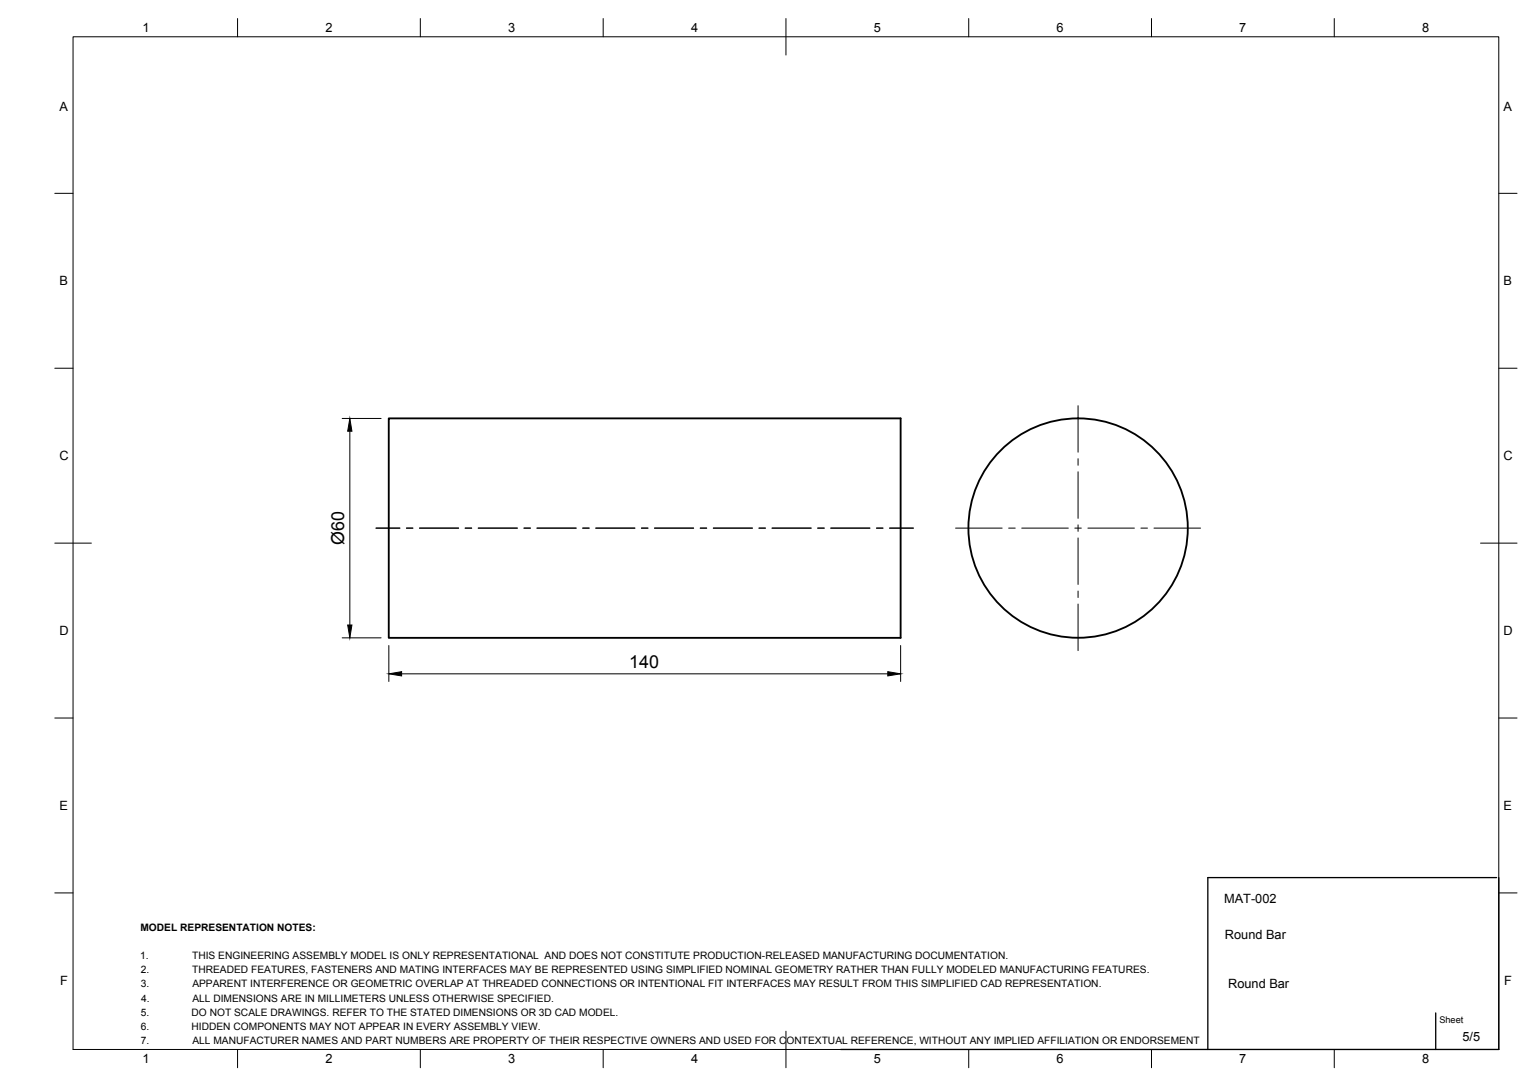
ISO-10303-21;
HEADER;
/* Generated by software containing ST-Developer
 * from STEP Tools, Inc. (www.steptools.com) 
 */

FILE_DESCRIPTION(
/* description */ ('STEP AP214'),
/* implementation_level */ '2;1');

FILE_NAME(
/* name */ 'Round Bar.step',
/* time_stamp */ '2026-11-14T04:35:10-08:00',
/* author */ (''),
/* organization */ (''),
/* preprocessor_version */ 'ST-DEVELOPER v20.2',
/* originating_system */ 'Autodesk Translation Framework v15.17.0.0',
/* authorisation */ '');

FILE_SCHEMA (('AUTOMOTIVE_DESIGN { 1 0 10303 214 3 1 1 }'));
ENDSEC;

DATA;
#10=MECHANICAL_DESIGN_GEOMETRIC_PRESENTATION_REPRESENTATION('',(#109),#2477);
#65=CIRCLE('',#1547,30.);
#66=CIRCLE('',#1548,30.);
#96=CYLINDRICAL_SURFACE('',#1546,30.);
#101=SHAPE_REPRESENTATION_RELATIONSHIP('SRR','None',#2499,#105);
#105=ADVANCED_BREP_SHAPE_REPRESENTATION('',(#113),#2475);
#109=STYLED_ITEM('',(#2528),#113);
#113=MANIFOLD_SOLID_BREP('Body1',#1429);
#166=FACE_OUTER_BOUND('',#247,.T.);
#167=FACE_OUTER_BOUND('',#248,.T.);
#168=FACE_OUTER_BOUND('',#249,.T.);
#247=EDGE_LOOP('',(#1178,#1179,#1180,#1181));
#248=EDGE_LOOP('',(#1182));
#249=EDGE_LOOP('',(#1183));
#401=LINE('',#2326,#548);
#548=VECTOR('',#1869,30.);
#665=VERTEX_POINT('',#2323);
#666=VERTEX_POINT('',#2325);
#839=EDGE_CURVE('',#665,#665,#65,.T.);
#840=EDGE_CURVE('',#665,#666,#401,.T.);
#841=EDGE_CURVE('',#666,#666,#66,.T.);
#1178=ORIENTED_EDGE('',*,*,#839,.F.);
#1179=ORIENTED_EDGE('',*,*,#840,.T.);
#1180=ORIENTED_EDGE('',*,*,#841,.T.);
#1181=ORIENTED_EDGE('',*,*,#840,.F.);
#1182=ORIENTED_EDGE('',*,*,#841,.F.);
#1183=ORIENTED_EDGE('',*,*,#839,.T.);
#1331=PLANE('',#1549);
#1332=PLANE('',#1550);
#1399=ADVANCED_FACE('',(#166),#96,.T.);
#1400=ADVANCED_FACE('',(#167),#1331,.F.);
#1401=ADVANCED_FACE('',(#168),#1332,.T.);
#1429=CLOSED_SHELL('',(#1399,#1400,#1401));
#1545=AXIS2_PLACEMENT_3D('',#2321,#1863,#1864);
#1546=AXIS2_PLACEMENT_3D('',#2322,#1865,#1866);
#1547=AXIS2_PLACEMENT_3D('',#2324,#1867,#1868);
#1548=AXIS2_PLACEMENT_3D('',#2327,#1870,#1871);
#1549=AXIS2_PLACEMENT_3D('',#2328,#1872,#1873);
#1550=AXIS2_PLACEMENT_3D('',#2329,#1874,#1875);
#1863=DIRECTION('axis',(0.,0.,1.));
#1864=DIRECTION('refdir',(1.,0.,0.));
#1865=DIRECTION('center_axis',(0.,0.,1.));
#1866=DIRECTION('ref_axis',(1.,0.,0.));
#1867=DIRECTION('center_axis',(0.,0.,1.));
#1868=DIRECTION('ref_axis',(1.,0.,0.));
#1869=DIRECTION('',(0.,0.,-1.));
#1870=DIRECTION('center_axis',(0.,0.,1.));
#1871=DIRECTION('ref_axis',(1.,0.,0.));
#1872=DIRECTION('center_axis',(0.,0.,1.));
#1873=DIRECTION('ref_axis',(1.,0.,0.));
#1874=DIRECTION('center_axis',(0.,0.,1.));
#1875=DIRECTION('ref_axis',(1.,0.,0.));
#2321=CARTESIAN_POINT('',(0.,0.,0.));
#2322=CARTESIAN_POINT('Origin',(-3.0679035930424E-16,0.,-105.));
#2323=CARTESIAN_POINT('',(-30.,-3.67394039744206E-15,35.));
#2324=CARTESIAN_POINT('Origin',(-3.0679035930424E-16,0.,35.));
#2325=CARTESIAN_POINT('',(-30.,-3.67394039744206E-15,-105.));
#2326=CARTESIAN_POINT('',(-30.,-3.67394039744206E-15,-105.));
#2327=CARTESIAN_POINT('Origin',(-3.0679035930424E-16,0.,-105.));
#2328=CARTESIAN_POINT('Origin',(-3.0679035930424E-16,0.,-105.));
#2329=CARTESIAN_POINT('Origin',(-3.0679035930424E-16,0.,35.));
#2469=UNCERTAINTY_MEASURE_WITH_UNIT(LENGTH_MEASURE(0.01),#2478,
'DISTANCE_ACCURACY_VALUE',
'Maximum model space distance between geometric entities at asserted c
onnectivities');
#2471=UNCERTAINTY_MEASURE_WITH_UNIT(LENGTH_MEASURE(0.01),#2478,
'DISTANCE_ACCURACY_VALUE',
'Maximum model space distance between geometric entities at asserted c
onnectivities');
#2475=(
GEOMETRIC_REPRESENTATION_CONTEXT(3)
GLOBAL_UNCERTAINTY_ASSIGNED_CONTEXT((#2469))
GLOBAL_UNIT_ASSIGNED_CONTEXT((#2478,#2480,#2481))
REPRESENTATION_CONTEXT('','3D')
);
#2477=(
GEOMETRIC_REPRESENTATION_CONTEXT(3)
GLOBAL_UNCERTAINTY_ASSIGNED_CONTEXT((#2471))
GLOBAL_UNIT_ASSIGNED_CONTEXT((#2478,#2480,#2481))
REPRESENTATION_CONTEXT('','3D')
);
#2478=(
LENGTH_UNIT()
NAMED_UNIT(*)
SI_UNIT(.MILLI.,.METRE.)
);
#2480=(
NAMED_UNIT(*)
PLANE_ANGLE_UNIT()
SI_UNIT($,.RADIAN.)
);
#2481=(
NAMED_UNIT(*)
SI_UNIT($,.STERADIAN.)
SOLID_ANGLE_UNIT()
);
#2485=SHAPE_DEFINITION_REPRESENTATION(#2490,#2499);
#2490=PRODUCT_DEFINITION_SHAPE('',$,#2505);
#2499=SHAPE_REPRESENTATION('',(#1545),#2475);
#2501=PRODUCT_DEFINITION_CONTEXT('part definition',#2518,'design');
#2505=PRODUCT_DEFINITION('Round Bar','Round Bar',#2510,#2501);
#2510=PRODUCT_DEFINITION_FORMATION('',$,#2523);
#2518=APPLICATION_CONTEXT(
'Core Data for Automotive Mechanical Design Process');
#2519=PRODUCT_CONTEXT('part definition',#2518,'mechanical');
#2523=PRODUCT('Round Bar','Round Bar',$,(#2519));
#2528=PRESENTATION_STYLE_ASSIGNMENT((#2533));
#2533=SURFACE_STYLE_USAGE(.BOTH.,#2538);
#2538=SURFACE_SIDE_STYLE('',(#2543));
#2543=SURFACE_STYLE_FILL_AREA(#2548);
#2548=FILL_AREA_STYLE('Opaque(227,224,212)',(#2553));
#2553=FILL_AREA_STYLE_COLOUR('Opaque(227,224,212)',#2558);
#2558=COLOUR_RGB('Opaque(227,224,212)',0.890196078431372,0.87843137254902,
0.831372549019608);
ENDSEC;
END-ISO-10303-21;
